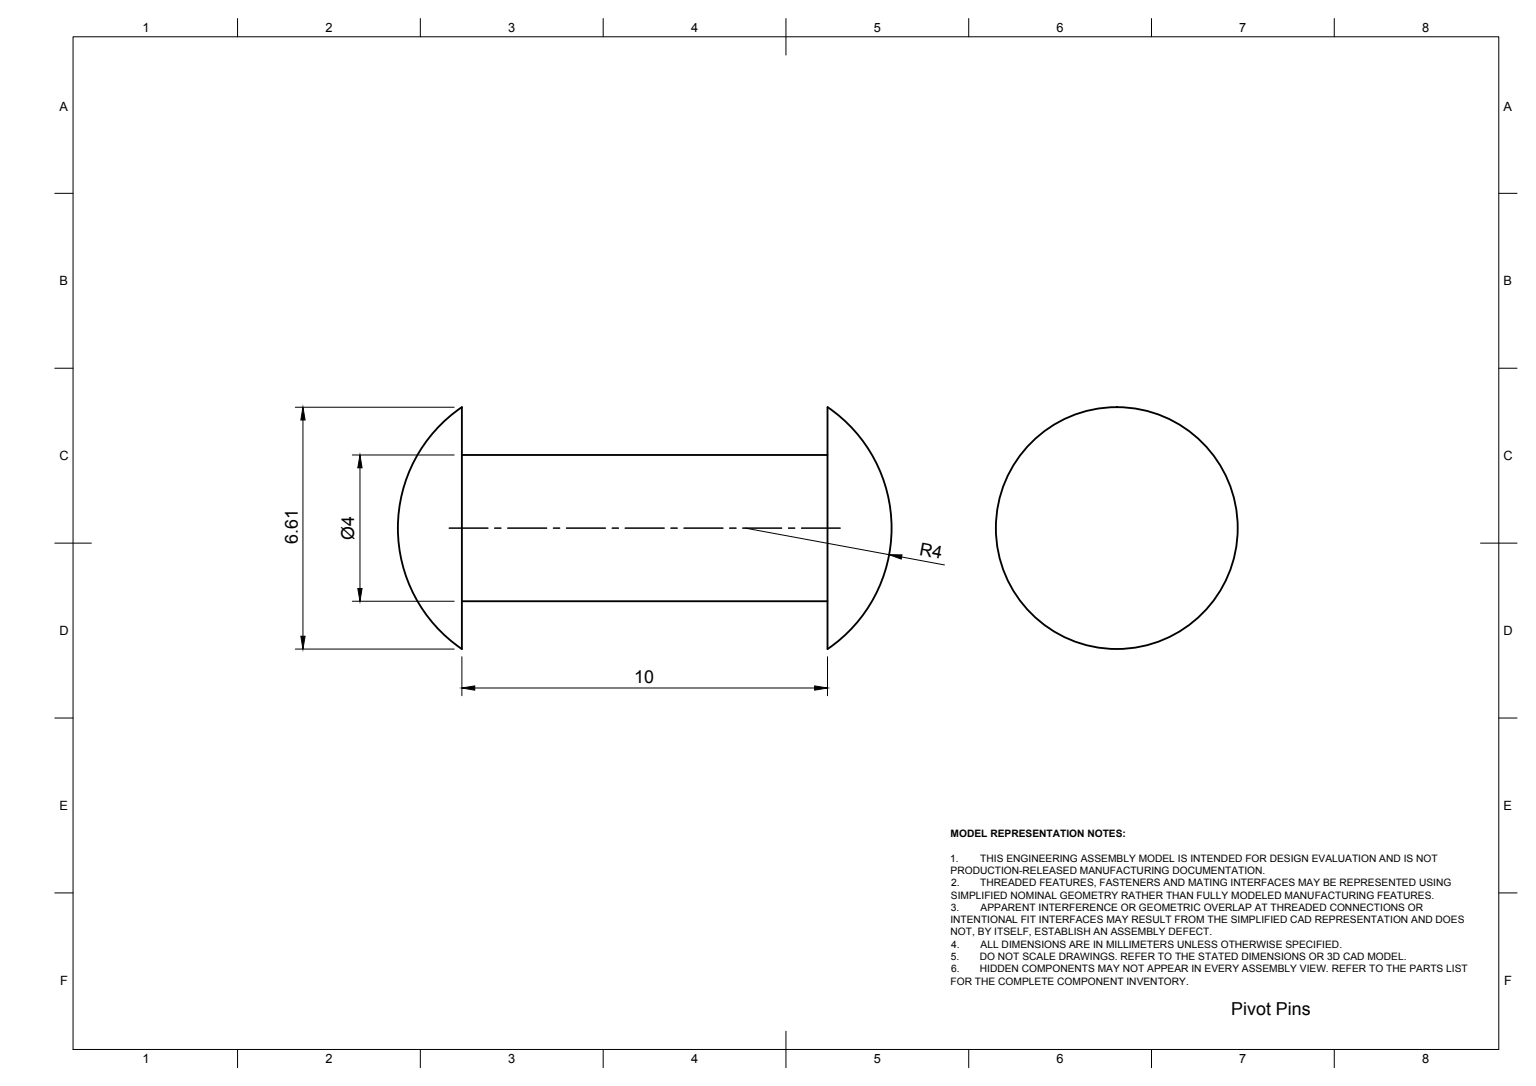
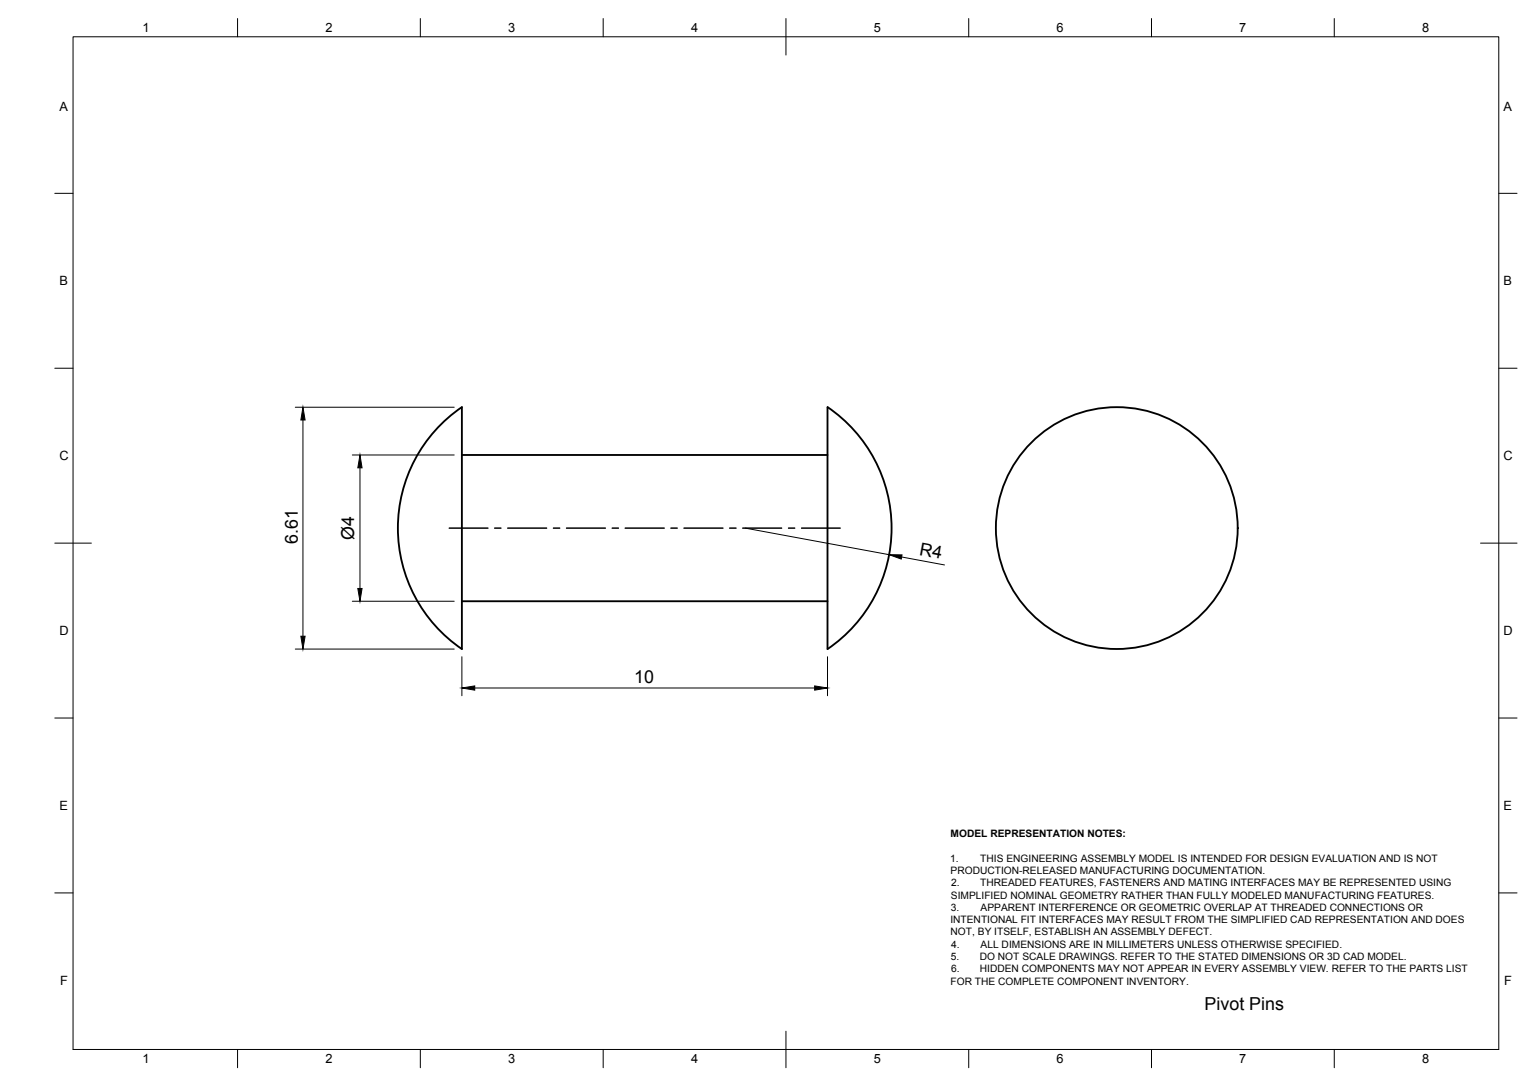
ISO-10303-21;
HEADER;
/* Generated by software containing ST-Developer
 * from STEP Tools, Inc. (www.steptools.com) 
 */

FILE_DESCRIPTION(
/* description */ ('STEP AP214'),
/* implementation_level */ '2;1');

FILE_NAME(
/* name */ 'Pivot Pins.step',
/* time_stamp */ '2026-10-06T11:11:25-07:00',
/* author */ (''),
/* organization */ (''),
/* preprocessor_version */ 'ST-DEVELOPER v20.2',
/* originating_system */ 'Autodesk Translation Framework v15.15.0.0',
/* authorisation */ '');

FILE_SCHEMA (('AUTOMOTIVE_DESIGN { 1 0 10303 214 3 1 1 }'));
ENDSEC;

DATA;
#10=MECHANICAL_DESIGN_GEOMETRIC_PRESENTATION_REPRESENTATION('',(#698),#47717);
#674=SHAPE_REPRESENTATION_RELATIONSHIP('SRR','None',#47761,#686);
#686=ADVANCED_BREP_SHAPE_REPRESENTATION('',(#710),#47705);
#698=STYLED_ITEM('',(#47830),#710);
#710=MANIFOLD_SOLID_BREP('Body1',#8925);
#722=FACE_BOUND('',#2579,.T.);
#723=FACE_BOUND('',#2581,.T.);
#759=PLANE('',#9079);
#760=PLANE('',#9080);
#883=LINE('',#12224,#1370);
#1370=VECTOR('',#9968,2.);
#1857=CYLINDRICAL_SURFACE('',#9074,2.);
#2063=FACE_OUTER_BOUND('',#2575,.T.);
#2064=FACE_OUTER_BOUND('',#2576,.T.);
#2065=FACE_OUTER_BOUND('',#2577,.T.);
#2066=FACE_OUTER_BOUND('',#2578,.T.);
#2067=FACE_OUTER_BOUND('',#2580,.T.);
#2575=EDGE_LOOP('',(#5727));
#2576=EDGE_LOOP('',(#5728,#5729,#5730,#5731));
#2577=EDGE_LOOP('',(#5732));
#2578=EDGE_LOOP('',(#5733));
#2579=EDGE_LOOP('',(#5734));
#2580=EDGE_LOOP('',(#5735));
#2581=EDGE_LOOP('',(#5736));
#3124=CIRCLE('',#9073,3.30718913883074);
#3125=CIRCLE('',#9075,2.);
#3126=CIRCLE('',#9076,2.);
#3127=CIRCLE('',#9078,3.30718913883074);
#3532=VERTEX_POINT('',#12218);
#3533=VERTEX_POINT('',#12221);
#3534=VERTEX_POINT('',#12223);
#3535=VERTEX_POINT('',#12227);
#4389=EDGE_CURVE('',#3532,#3532,#3124,.T.);
#4390=EDGE_CURVE('',#3533,#3533,#3125,.T.);
#4391=EDGE_CURVE('',#3533,#3534,#883,.T.);
#4392=EDGE_CURVE('',#3534,#3534,#3126,.T.);
#4393=EDGE_CURVE('',#3535,#3535,#3127,.T.);
#5727=ORIENTED_EDGE('',*,*,#4389,.T.);
#5728=ORIENTED_EDGE('',*,*,#4390,.F.);
#5729=ORIENTED_EDGE('',*,*,#4391,.T.);
#5730=ORIENTED_EDGE('',*,*,#4392,.T.);
#5731=ORIENTED_EDGE('',*,*,#4391,.F.);
#5732=ORIENTED_EDGE('',*,*,#4393,.F.);
#5733=ORIENTED_EDGE('',*,*,#4393,.T.);
#5734=ORIENTED_EDGE('',*,*,#4392,.F.);
#5735=ORIENTED_EDGE('',*,*,#4389,.F.);
#5736=ORIENTED_EDGE('',*,*,#4390,.T.);
#8403=SPHERICAL_SURFACE('',#9072,4.);
#8404=SPHERICAL_SURFACE('',#9077,4.);
#8413=ADVANCED_FACE('',(#2063),#8403,.T.);
#8414=ADVANCED_FACE('',(#2064),#1857,.T.);
#8415=ADVANCED_FACE('',(#2065),#8404,.T.);
#8416=ADVANCED_FACE('',(#2066,#722),#759,.T.);
#8417=ADVANCED_FACE('',(#2067,#723),#760,.T.);
#8925=CLOSED_SHELL('',(#8413,#8414,#8415,#8416,#8417));
#9071=AXIS2_PLACEMENT_3D('',#12216,#9958,#9959);
#9072=AXIS2_PLACEMENT_3D('',#12217,#9960,#9961);
#9073=AXIS2_PLACEMENT_3D('',#12219,#9962,#9963);
#9074=AXIS2_PLACEMENT_3D('',#12220,#9964,#9965);
#9075=AXIS2_PLACEMENT_3D('',#12222,#9966,#9967);
#9076=AXIS2_PLACEMENT_3D('',#12225,#9969,#9970);
#9077=AXIS2_PLACEMENT_3D('',#12226,#9971,#9972);
#9078=AXIS2_PLACEMENT_3D('',#12228,#9973,#9974);
#9079=AXIS2_PLACEMENT_3D('',#12229,#9975,#9976);
#9080=AXIS2_PLACEMENT_3D('',#12230,#9977,#9978);
#9958=DIRECTION('axis',(0.,0.,1.));
#9959=DIRECTION('refdir',(1.,0.,0.));
#9960=DIRECTION('center_axis',(0.,-1.,0.));
#9961=DIRECTION('ref_axis',(1.,0.,0.));
#9962=DIRECTION('center_axis',(2.50063434304147E-17,1.27632226958495E-16,
1.));
#9963=DIRECTION('ref_axis',(3.19161530011276E-33,-1.,1.27632226958495E-16));
#9964=DIRECTION('center_axis',(2.50063434304147E-17,1.27632226958495E-16,
1.));
#9965=DIRECTION('ref_axis',(3.19161530011276E-33,-1.,1.27632226958495E-16));
#9966=DIRECTION('center_axis',(2.50063434304147E-17,1.27632226958495E-16,
1.));
#9967=DIRECTION('ref_axis',(3.19161530011276E-33,-1.,1.27632226958495E-16));
#9968=DIRECTION('',(-2.50063434304147E-17,-1.27632226958495E-16,-1.));
#9969=DIRECTION('center_axis',(2.50063434304147E-17,1.27632226958495E-16,
1.));
#9970=DIRECTION('ref_axis',(3.19161530011276E-33,-1.,1.27632226958495E-16));
#9971=DIRECTION('center_axis',(0.,1.,0.));
#9972=DIRECTION('ref_axis',(1.,0.,0.));
#9973=DIRECTION('center_axis',(2.50063434304147E-17,1.27632226958495E-16,
1.));
#9974=DIRECTION('ref_axis',(3.19161530011276E-33,-1.,1.27632226958495E-16));
#9975=DIRECTION('center_axis',(2.50063434304147E-17,1.27632226958495E-16,
1.));
#9976=DIRECTION('ref_axis',(2.50063434304147E-17,-1.,1.27632226958495E-16));
#9977=DIRECTION('center_axis',(-2.50063434304147E-17,-1.27632226958495E-16,
-1.));
#9978=DIRECTION('ref_axis',(2.50063434304147E-17,-1.,1.27632226958495E-16));
#12216=CARTESIAN_POINT('',(0.,0.,0.));
#12217=CARTESIAN_POINT('Origin',(-69.9391102914976,14.1820463536523,178.735485069079));
#12218=CARTESIAN_POINT('',(-73.2462994303283,14.1820463536523,180.985485069079));
#12219=CARTESIAN_POINT('Origin',(-69.9391102914976,14.1820463536523,180.985485069079));
#12220=CARTESIAN_POINT('Origin',(-69.9391102914976,14.1820463536523,175.985485069079));
#12221=CARTESIAN_POINT('',(-69.9391102914976,16.1820463536523,180.985485069079));
#12222=CARTESIAN_POINT('Origin',(-69.9391102914976,14.1820463536523,180.985485069079));
#12223=CARTESIAN_POINT('',(-69.9391102914976,16.1820463536523,170.985485069079));
#12224=CARTESIAN_POINT('',(-69.9391102914976,16.1820463536523,175.985485069079));
#12225=CARTESIAN_POINT('Origin',(-69.9391102914976,14.1820463536523,170.985485069079));
#12226=CARTESIAN_POINT('Origin',(-69.9391102914976,14.1820463536523,173.235485069079));
#12227=CARTESIAN_POINT('',(-73.2462994303283,14.1820463536523,170.985485069079));
#12228=CARTESIAN_POINT('Origin',(-69.9391102914976,14.1820463536523,170.985485069079));
#12229=CARTESIAN_POINT('Origin',(-67.9391102914976,14.1820463536523,170.985485069079));
#12230=CARTESIAN_POINT('Origin',(-67.9391102914976,14.1820463536523,180.985485069079));
#47691=UNCERTAINTY_MEASURE_WITH_UNIT(LENGTH_MEASURE(0.01),#47718,
'DISTANCE_ACCURACY_VALUE',
'Maximum model space distance between geometric entities at asserted c
onnectivities');
#47703=UNCERTAINTY_MEASURE_WITH_UNIT(LENGTH_MEASURE(0.01),#47718,
'DISTANCE_ACCURACY_VALUE',
'Maximum model space distance between geometric entities at asserted c
onnectivities');
#47705=(
GEOMETRIC_REPRESENTATION_CONTEXT(3)
GLOBAL_UNCERTAINTY_ASSIGNED_CONTEXT((#47691))
GLOBAL_UNIT_ASSIGNED_CONTEXT((#47718,#47720,#47721))
REPRESENTATION_CONTEXT('','3D')
);
#47717=(
GEOMETRIC_REPRESENTATION_CONTEXT(3)
GLOBAL_UNCERTAINTY_ASSIGNED_CONTEXT((#47703))
GLOBAL_UNIT_ASSIGNED_CONTEXT((#47718,#47720,#47721))
REPRESENTATION_CONTEXT('','3D')
);
#47718=(
LENGTH_UNIT()
NAMED_UNIT(*)
SI_UNIT(.MILLI.,.METRE.)
);
#47720=(
NAMED_UNIT(*)
PLANE_ANGLE_UNIT()
SI_UNIT($,.RADIAN.)
);
#47721=(
NAMED_UNIT(*)
SI_UNIT($,.STERADIAN.)
SOLID_ANGLE_UNIT()
);
#47723=SHAPE_DEFINITION_REPRESENTATION(#47736,#47761);
#47736=PRODUCT_DEFINITION_SHAPE('',$,#47775);
#47761=SHAPE_REPRESENTATION('',(#9071),#47705);
#47773=PRODUCT_DEFINITION_CONTEXT('part definition',#47814,'design');
#47775=PRODUCT_DEFINITION('Pivot Pins','Pivot Pins',#47788,#47773);
#47788=PRODUCT_DEFINITION_FORMATION('',$,#47817);
#47814=APPLICATION_CONTEXT(
'Core Data for Automotive Mechanical Design Process');
#47815=PRODUCT_CONTEXT('part definition',#47814,'mechanical');
#47817=PRODUCT('Pivot Pins','Pivot Pins',$,(#47815));
#47830=PRESENTATION_STYLE_ASSIGNMENT((#47832));
#47832=SURFACE_STYLE_USAGE(.BOTH.,#47834);
#47834=SURFACE_SIDE_STYLE('',(#47836));
#47836=SURFACE_STYLE_FILL_AREA(#47838);
#47838=FILL_AREA_STYLE('Opaque(202,209,238)',(#47840));
#47840=FILL_AREA_STYLE_COLOUR('Opaque(202,209,238)',#47842);
#47842=COLOUR_RGB('Opaque(202,209,238)', 0.66274510, 0.83137255, 0.94901961);
ENDSEC;
END-ISO-10303-21;
